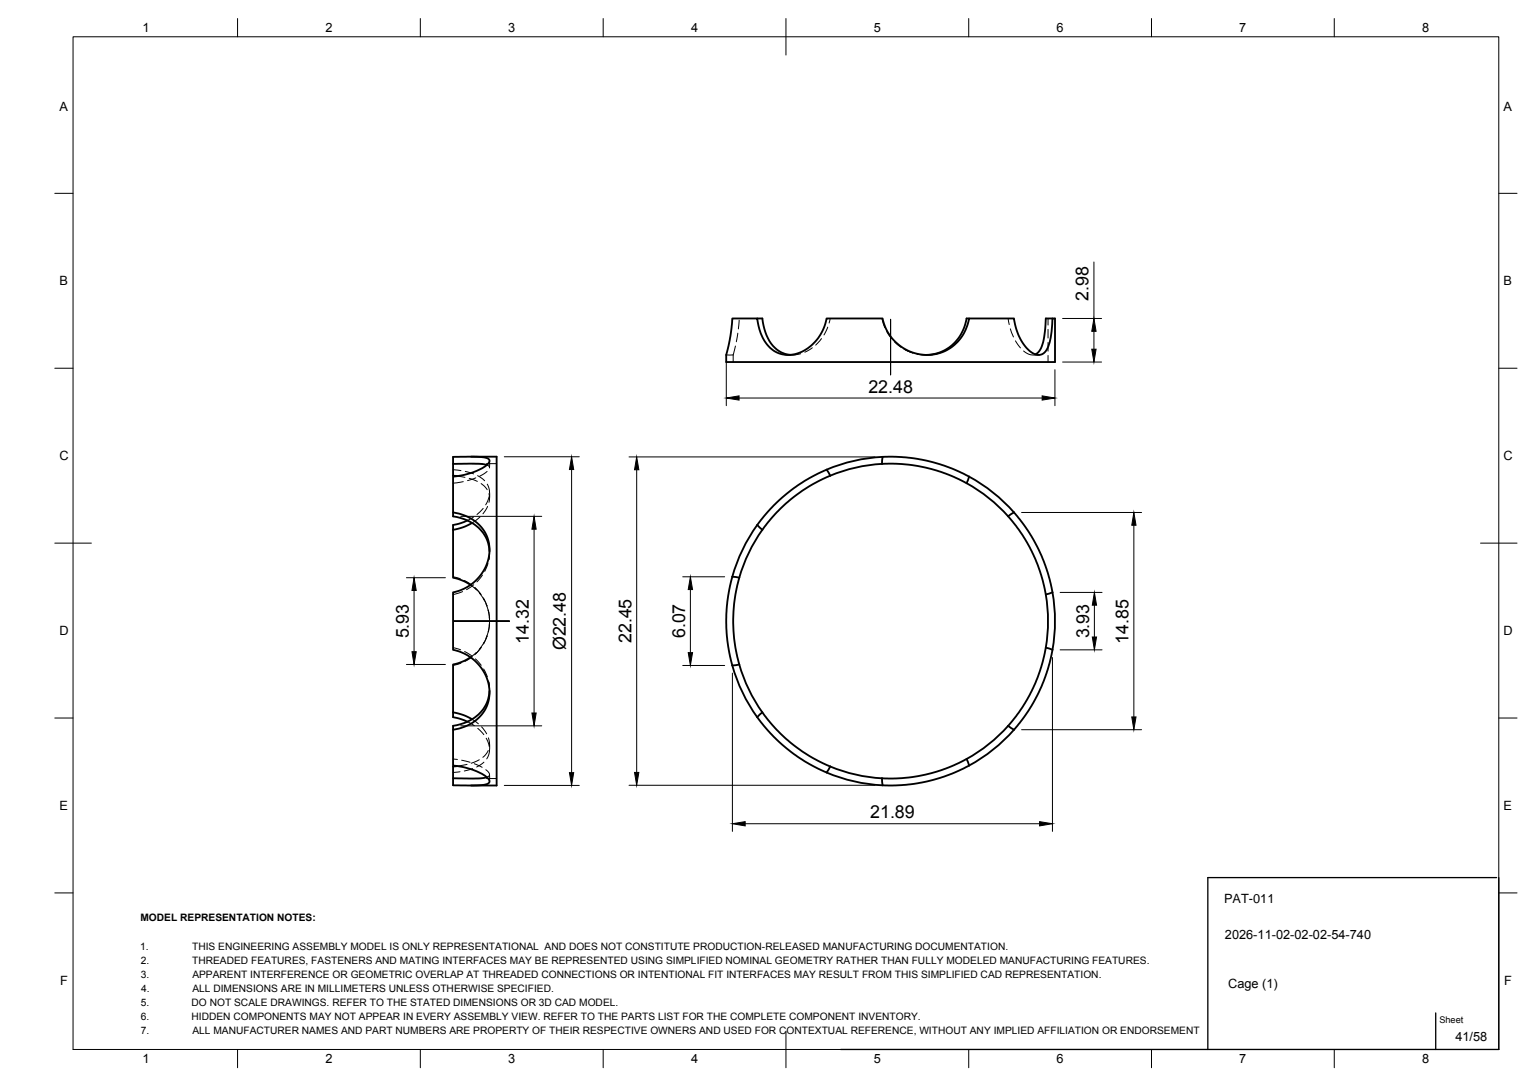
ISO-10303-21;
HEADER;
/* Generated by software containing ST-Developer
 * from STEP Tools, Inc. (www.steptools.com) 
 */

FILE_DESCRIPTION(
/* description */ ('Belt tension measurement rig'),
/* implementation_level */ '2;1');

FILE_NAME(
/* name */ 'Cage (1).step',
/* time_stamp */ '2026-10-28T03:24:44-07:00',
/* author */ (''),
/* organization */ (''),
/* preprocessor_version */ 'ST-DEVELOPER v20.2',
/* originating_system */ 'Autodesk Translation Framework v15.17.0.0',
/* authorisation */ '');

FILE_SCHEMA (('AUTOMOTIVE_DESIGN { 1 0 10303 214 3 1 1 }'));
ENDSEC;

DATA;
#10=MECHANICAL_DESIGN_GEOMETRIC_PRESENTATION_REPRESENTATION('',(#740),#23587);
#460=SPHERICAL_SURFACE('',#13710,0.309556);
#461=SPHERICAL_SURFACE('',#13726,0.309556);
#462=SPHERICAL_SURFACE('',#13731,0.309556);
#463=SPHERICAL_SURFACE('',#13737,0.309556);
#464=SPHERICAL_SURFACE('',#13742,0.309556);
#465=SPHERICAL_SURFACE('',#13747,0.309556);
#466=SPHERICAL_SURFACE('',#13755,0.309556);
#517=B_SPLINE_CURVE_WITH_KNOTS('',3,(#20953,#20954,#20955,#20956,#20957,
#20958,#20959,#20960,#20961,#20962,#20963,#20964,#20965,#20966,#20967,#20968,
#20969,#20970,#20971,#20972,#20973,#20974),.UNSPECIFIED.,.F.,.F.,(4,2,2,
2,2,2,2,2,2,2,4),(0.0591825211272536,0.157966726598481,0.236950089897721,
0.315933453196962,0.391576304923761,0.46721915665056,0.54286200837736,0.618504860104159,
0.697488223403399,0.77647158670264,0.875255792173867),.UNSPECIFIED.);
#518=B_SPLINE_CURVE_WITH_KNOTS('',3,(#20978,#20979,#20980,#20981,#20982,
#20983,#20984,#20985,#20986,#20987,#20988,#20989,#20990,#20991,#20992,#20993,
#20994,#20995,#20996,#20997,#20998,#20999),.UNSPECIFIED.,.F.,.F.,(4,2,2,
2,2,2,2,2,2,2,4),(0.0581119756758434,0.106553146291161,0.213106292582322,
0.30849933801665,0.386091982889075,0.4636846277615,0.541277272633925,0.61886991750635,
0.714262962940678,0.820816109231839,0.869257279847157),.UNSPECIFIED.);
#519=B_SPLINE_CURVE_WITH_KNOTS('',3,(#21005,#21006,#21007,#21008,#21009,
#21010,#21011,#21012,#21013,#21014,#21015,#21016,#21017,#21018,#21019,#21020,
#21021,#21022,#21023,#21024,#21025,#21026),.UNSPECIFIED.,.F.,.F.,(4,2,2,
2,2,2,2,2,2,2,4),(0.0581119756758434,0.106553146291161,0.213106292582322,
0.30849933801665,0.386091982889075,0.4636846277615,0.541277272633925,0.61886991750635,
0.714262962940679,0.820816109231839,0.869257279847157),.UNSPECIFIED.);
#520=B_SPLINE_CURVE_WITH_KNOTS('',3,(#21030,#21031,#21032,#21033,#21034,
#21035,#21036,#21037,#21038,#21039,#21040,#21041,#21042,#21043,#21044,#21045,
#21046,#21047,#21048,#21049,#21050,#21051),.UNSPECIFIED.,.F.,.F.,(4,2,2,
2,2,2,2,2,2,2,4),(0.0581119756758433,0.106553146291161,0.213106292582322,
0.308499338016649,0.386091982889075,0.4636846277615,0.541277272633925,0.61886991750635,
0.714262962940678,0.820816109231839,0.869257279847157),.UNSPECIFIED.);
#521=B_SPLINE_CURVE_WITH_KNOTS('',3,(#21060,#21061,#21062,#21063,#21064,
#21065,#21066,#21067,#21068,#21069,#21070,#21071,#21072,#21073,#21074,#21075,
#21076,#21077,#21078,#21079,#21080,#21081),.UNSPECIFIED.,.F.,.F.,(4,2,2,
2,2,2,2,2,2,2,4),(0.0581119756758433,0.106553146291161,0.213106292582322,
0.30849933801665,0.386091982889075,0.4636846277615,0.541277272633925,0.61886991750635,
0.714262962940678,0.820816109231839,0.869257279847157),.UNSPECIFIED.);
#522=B_SPLINE_CURVE_WITH_KNOTS('',3,(#21085,#21086,#21087,#21088,#21089,
#21090,#21091,#21092,#21093,#21094,#21095,#21096,#21097,#21098,#21099,#21100,
#21101,#21102,#21103,#21104,#21105,#21106),.UNSPECIFIED.,.F.,.F.,(4,2,2,
2,2,2,2,2,2,2,4),(0.0581119756758434,0.106553146291161,0.213106292582322,
0.30849933801665,0.386091982889075,0.4636846277615,0.541277272633925,0.61886991750635,
0.714262962940678,0.820816109231839,0.869257279847157),.UNSPECIFIED.);
#523=B_SPLINE_CURVE_WITH_KNOTS('',3,(#21110,#21111,#21112,#21113,#21114,
#21115,#21116,#21117,#21118,#21119,#21120,#21121,#21122,#21123,#21124,#21125,
#21126,#21127,#21128,#21129,#21130,#21131),.UNSPECIFIED.,.F.,.F.,(4,2,2,
2,2,2,2,2,2,2,4),(0.0581119756758434,0.106553146291161,0.213106292582322,
0.30849933801665,0.386091982889075,0.4636846277615,0.541277272633925,0.61886991750635,
0.714262962940678,0.820816109231839,0.869257279847157),.UNSPECIFIED.);
#524=B_SPLINE_CURVE_WITH_KNOTS('',3,(#21135,#21136,#21137,#21138,#21139,
#21140,#21141,#21142,#21143,#21144,#21145,#21146,#21147,#21148,#21149,#21150,
#21151,#21152,#21153,#21154,#21155,#21156),.UNSPECIFIED.,.F.,.F.,(4,2,2,
2,2,2,2,2,2,2,4),(0.0581119756758433,0.106553146291161,0.213106292582322,
0.30849933801665,0.386091982889075,0.4636846277615,0.541277272633925,0.61886991750635,
0.714262962940678,0.820816109231839,0.869257279847157),.UNSPECIFIED.);
#525=B_SPLINE_CURVE_WITH_KNOTS('',3,(#21164,#21165,#21166,#21167,#21168,
#21169,#21170,#21171,#21172,#21173,#21174,#21175,#21176,#21177,#21178,#21179,
#21180,#21181,#21182,#21183,#21184,#21185),.UNSPECIFIED.,.F.,.F.,(4,2,2,
2,2,2,2,2,2,2,4),(0.0591825211272536,0.157966726598481,0.236950089897721,
0.315933453196962,0.391576304923761,0.467219156650561,0.54286200837736,
0.618504860104159,0.697488223403399,0.77647158670264,0.875255792173867),
 .UNSPECIFIED.);
#526=B_SPLINE_CURVE_WITH_KNOTS('',3,(#21193,#21194,#21195,#21196,#21197,
#21198,#21199,#21200,#21201,#21202,#21203,#21204,#21205,#21206,#21207,#21208,
#21209,#21210,#21211,#21212,#21213,#21214),.UNSPECIFIED.,.F.,.F.,(4,2,2,
2,2,2,2,2,2,2,4),(0.0591825211272536,0.157966726598481,0.236950089897722,
0.315933453196962,0.391576304923761,0.467219156650561,0.54286200837736,
0.618504860104159,0.697488223403399,0.77647158670264,0.875255792173867),
 .UNSPECIFIED.);
#527=B_SPLINE_CURVE_WITH_KNOTS('',3,(#21224,#21225,#21226,#21227,#21228,
#21229,#21230,#21231,#21232,#21233,#21234,#21235,#21236,#21237,#21238,#21239,
#21240,#21241,#21242,#21243,#21244,#21245),.UNSPECIFIED.,.F.,.F.,(4,2,2,
2,2,2,2,2,2,2,4),(0.0591825211272536,0.157966726598481,0.236950089897721,
0.315933453196962,0.391576304923761,0.46721915665056,0.54286200837736,0.618504860104159,
0.697488223403399,0.77647158670264,0.875255792173867),.UNSPECIFIED.);
#528=B_SPLINE_CURVE_WITH_KNOTS('',3,(#21253,#21254,#21255,#21256,#21257,
#21258,#21259,#21260,#21261,#21262,#21263,#21264,#21265,#21266,#21267,#21268,
#21269,#21270,#21271,#21272,#21273,#21274),.UNSPECIFIED.,.F.,.F.,(4,2,2,
2,2,2,2,2,2,2,4),(0.0591825211272536,0.157966726598481,0.236950089897721,
0.315933453196962,0.391576304923761,0.46721915665056,0.542862008377359,
0.618504860104159,0.697488223403399,0.776471586702639,0.875255792173867),
 .UNSPECIFIED.);
#529=B_SPLINE_CURVE_WITH_KNOTS('',3,(#21282,#21283,#21284,#21285,#21286,
#21287,#21288,#21289,#21290,#21291,#21292,#21293,#21294,#21295,#21296,#21297,
#21298,#21299,#21300,#21301,#21302,#21303),.UNSPECIFIED.,.F.,.F.,(4,2,2,
2,2,2,2,2,2,2,4),(0.0591825211272536,0.157966726598481,0.236950089897721,
0.315933453196962,0.391576304923761,0.46721915665056,0.54286200837736,0.618504860104159,
0.697488223403399,0.77647158670264,0.875255792173867),.UNSPECIFIED.);
#530=B_SPLINE_CURVE_WITH_KNOTS('',3,(#21312,#21313,#21314,#21315,#21316,
#21317,#21318,#21319,#21320,#21321,#21322,#21323,#21324,#21325,#21326,#21327,
#21328,#21329,#21330,#21331,#21332,#21333),.UNSPECIFIED.,.F.,.F.,(4,2,2,
2,2,2,2,2,2,2,4),(0.0591825211272536,0.157966726598481,0.236950089897721,
0.315933453196962,0.391576304923761,0.46721915665056,0.542862008377359,
0.618504860104159,0.697488223403399,0.776471586702639,0.875255792173867),
 .UNSPECIFIED.);
#616=SHAPE_REPRESENTATION_RELATIONSHIP('SRR','None',#23865,#671);
#671=ADVANCED_BREP_SHAPE_REPRESENTATION('',(#809),#23563);
#740=STYLED_ITEM('',(#24211),#809);
#809=MANIFOLD_SOLID_BREP('Continuous crown cage',#12246);
#978=FACE_BOUND('',#2627,.T.);
#1254=PLANE('',#13723);
#1255=PLANE('',#13728);
#1256=PLANE('',#13733);
#1257=PLANE('',#13739);
#1258=PLANE('',#13744);
#1259=PLANE('',#13753);
#1260=PLANE('',#13757);
#1261=PLANE('',#13758);
#1758=FACE_OUTER_BOUND('',#2611,.T.);
#1759=FACE_OUTER_BOUND('',#2612,.T.);
#1760=FACE_OUTER_BOUND('',#2613,.T.);
#1761=FACE_OUTER_BOUND('',#2614,.T.);
#1762=FACE_OUTER_BOUND('',#2615,.T.);
#1763=FACE_OUTER_BOUND('',#2616,.T.);
#1764=FACE_OUTER_BOUND('',#2617,.T.);
#1765=FACE_OUTER_BOUND('',#2618,.T.);
#1766=FACE_OUTER_BOUND('',#2619,.T.);
#1767=FACE_OUTER_BOUND('',#2620,.T.);
#1768=FACE_OUTER_BOUND('',#2621,.T.);
#1769=FACE_OUTER_BOUND('',#2622,.T.);
#1770=FACE_OUTER_BOUND('',#2623,.T.);
#1771=FACE_OUTER_BOUND('',#2624,.T.);
#1772=FACE_OUTER_BOUND('',#2625,.T.);
#1773=FACE_OUTER_BOUND('',#2626,.T.);
#1774=FACE_OUTER_BOUND('',#2628,.T.);
#2611=EDGE_LOOP('',(#9740,#9741,#9742,#9743));
#2612=EDGE_LOOP('',(#9744,#9745,#9746,#9747,#9748,#9749,#9750,#9751,#9752,
#9753,#9754,#9755,#9756,#9757,#9758,#9759,#9760,#9761));
#2613=EDGE_LOOP('',(#9762,#9763,#9764,#9765));
#2614=EDGE_LOOP('',(#9766,#9767,#9768,#9769));
#2615=EDGE_LOOP('',(#9770,#9771,#9772,#9773));
#2616=EDGE_LOOP('',(#9774,#9775,#9776,#9777));
#2617=EDGE_LOOP('',(#9778,#9779,#9780,#9781,#9782,#9783));
#2618=EDGE_LOOP('',(#9784,#9785,#9786,#9787));
#2619=EDGE_LOOP('',(#9788,#9789,#9790,#9791));
#2620=EDGE_LOOP('',(#9792,#9793,#9794,#9795));
#2621=EDGE_LOOP('',(#9796,#9797,#9798,#9799));
#2622=EDGE_LOOP('',(#9800,#9801,#9802,#9803));
#2623=EDGE_LOOP('',(#9804,#9805,#9806,#9807,#9808,#9809,#9810,#9811,#9812,
#9813,#9814,#9815,#9816,#9817,#9818,#9819,#9820,#9821));
#2624=EDGE_LOOP('',(#9822,#9823,#9824,#9825));
#2625=EDGE_LOOP('',(#9826,#9827,#9828,#9829));
#2626=EDGE_LOOP('',(#9830));
#2627=EDGE_LOOP('',(#9831));
#2628=EDGE_LOOP('',(#9832,#9833,#9834,#9835));
#3464=LINE('',#21055,#4215);
#3465=LINE('',#21308,#4216);
#4215=VECTOR('',#16695,1.123812);
#4216=VECTOR('',#16764,1.076188);
#4849=CIRCLE('',#13711,0.303778037777585);
#4850=CIRCLE('',#13712,0.303778037777585);
#4851=CIRCLE('',#13714,1.123812);
#4852=CIRCLE('',#13715,1.123812);
#4853=CIRCLE('',#13716,1.123812);
#4854=CIRCLE('',#13717,1.123812);
#4855=CIRCLE('',#13718,1.123812);
#4856=CIRCLE('',#13719,1.123812);
#4857=CIRCLE('',#13720,1.123812);
#4858=CIRCLE('',#13721,1.123812);
#4859=CIRCLE('',#13722,1.123812);
#4860=CIRCLE('',#13724,1.076188);
#4861=CIRCLE('',#13725,0.303778037777585);
#4862=CIRCLE('',#13727,0.303778037777585);
#4863=CIRCLE('',#13729,1.076188);
#4864=CIRCLE('',#13730,0.303778037777585);
#4865=CIRCLE('',#13732,0.303778037777585);
#4866=CIRCLE('',#13734,1.076188);
#4867=CIRCLE('',#13735,1.076188);
#4868=CIRCLE('',#13736,0.303778037777585);
#4869=CIRCLE('',#13738,0.303778037777585);
#4870=CIRCLE('',#13740,1.076188);
#4871=CIRCLE('',#13741,0.303778037777585);
#4872=CIRCLE('',#13743,0.303778037777585);
#4873=CIRCLE('',#13745,1.076188);
#4874=CIRCLE('',#13746,0.303778037777585);
#4875=CIRCLE('',#13748,0.303778037777585);
#4876=CIRCLE('',#13750,1.076188);
#4877=CIRCLE('',#13751,1.076188);
#4878=CIRCLE('',#13752,1.076188);
#4879=CIRCLE('',#13754,0.303778037777585);
#4880=CIRCLE('',#13756,0.303778037777585);
#5852=VERTEX_POINT('',#20951);
#5853=VERTEX_POINT('',#20952);
#5854=VERTEX_POINT('',#20975);
#5855=VERTEX_POINT('',#20977);
#5856=VERTEX_POINT('',#21002);
#5857=VERTEX_POINT('',#21004);
#5858=VERTEX_POINT('',#21027);
#5859=VERTEX_POINT('',#21029);
#5860=VERTEX_POINT('',#21052);
#5861=VERTEX_POINT('',#21054);
#5862=VERTEX_POINT('',#21057);
#5863=VERTEX_POINT('',#21059);
#5864=VERTEX_POINT('',#21082);
#5865=VERTEX_POINT('',#21084);
#5866=VERTEX_POINT('',#21107);
#5867=VERTEX_POINT('',#21109);
#5868=VERTEX_POINT('',#21132);
#5869=VERTEX_POINT('',#21134);
#5870=VERTEX_POINT('',#21159);
#5871=VERTEX_POINT('',#21163);
#5872=VERTEX_POINT('',#21188);
#5873=VERTEX_POINT('',#21192);
#5874=VERTEX_POINT('',#21217);
#5875=VERTEX_POINT('',#21219);
#5876=VERTEX_POINT('',#21223);
#5877=VERTEX_POINT('',#21248);
#5878=VERTEX_POINT('',#21252);
#5879=VERTEX_POINT('',#21277);
#5880=VERTEX_POINT('',#21281);
#5881=VERTEX_POINT('',#21306);
#5882=VERTEX_POINT('',#21309);
#5883=VERTEX_POINT('',#21311);
#7229=EDGE_CURVE('',#5852,#5853,#517,.T.);
#7230=EDGE_CURVE('',#5854,#5852,#4849,.T.);
#7231=EDGE_CURVE('',#5855,#5854,#518,.T.);
#7232=EDGE_CURVE('',#5853,#5855,#4850,.T.);
#7233=EDGE_CURVE('',#5856,#5854,#4851,.T.);
#7234=EDGE_CURVE('',#5856,#5857,#519,.T.);
#7235=EDGE_CURVE('',#5858,#5857,#4852,.T.);
#7236=EDGE_CURVE('',#5858,#5859,#520,.T.);
#7237=EDGE_CURVE('',#5860,#5859,#4853,.T.);
#7238=EDGE_CURVE('',#5860,#5861,#3464,.T.);
#7239=EDGE_CURVE('',#5861,#5861,#4854,.T.);
#7240=EDGE_CURVE('',#5862,#5860,#4855,.T.);
#7241=EDGE_CURVE('',#5862,#5863,#521,.T.);
#7242=EDGE_CURVE('',#5864,#5863,#4856,.T.);
#7243=EDGE_CURVE('',#5864,#5865,#522,.T.);
#7244=EDGE_CURVE('',#5866,#5865,#4857,.T.);
#7245=EDGE_CURVE('',#5866,#5867,#523,.T.);
#7246=EDGE_CURVE('',#5868,#5867,#4858,.T.);
#7247=EDGE_CURVE('',#5868,#5869,#524,.T.);
#7248=EDGE_CURVE('',#5855,#5869,#4859,.T.);
#7249=EDGE_CURVE('',#5852,#5870,#4860,.T.);
#7250=EDGE_CURVE('',#5870,#5856,#4861,.T.);
#7251=EDGE_CURVE('',#5871,#5870,#525,.T.);
#7252=EDGE_CURVE('',#5857,#5871,#4862,.T.);
#7253=EDGE_CURVE('',#5871,#5872,#4863,.T.);
#7254=EDGE_CURVE('',#5872,#5858,#4864,.T.);
#7255=EDGE_CURVE('',#5873,#5872,#526,.T.);
#7256=EDGE_CURVE('',#5859,#5873,#4865,.T.);
#7257=EDGE_CURVE('',#5873,#5874,#4866,.T.);
#7258=EDGE_CURVE('',#5874,#5875,#4867,.T.);
#7259=EDGE_CURVE('',#5875,#5862,#4868,.T.);
#7260=EDGE_CURVE('',#5876,#5875,#527,.T.);
#7261=EDGE_CURVE('',#5863,#5876,#4869,.T.);
#7262=EDGE_CURVE('',#5876,#5877,#4870,.T.);
#7263=EDGE_CURVE('',#5877,#5864,#4871,.T.);
#7264=EDGE_CURVE('',#5878,#5877,#528,.T.);
#7265=EDGE_CURVE('',#5865,#5878,#4872,.T.);
#7266=EDGE_CURVE('',#5878,#5879,#4873,.T.);
#7267=EDGE_CURVE('',#5879,#5866,#4874,.T.);
#7268=EDGE_CURVE('',#5880,#5879,#529,.T.);
#7269=EDGE_CURVE('',#5867,#5880,#4875,.T.);
#7270=EDGE_CURVE('',#5881,#5881,#4876,.T.);
#7271=EDGE_CURVE('',#5881,#5874,#3465,.T.);
#7272=EDGE_CURVE('',#5882,#5853,#4877,.T.);
#7273=EDGE_CURVE('',#5882,#5883,#530,.T.);
#7274=EDGE_CURVE('',#5880,#5883,#4878,.T.);
#7275=EDGE_CURVE('',#5869,#5882,#4879,.T.);
#7276=EDGE_CURVE('',#5883,#5868,#4880,.T.);
#9740=ORIENTED_EDGE('',*,*,#7229,.F.);
#9741=ORIENTED_EDGE('',*,*,#7230,.F.);
#9742=ORIENTED_EDGE('',*,*,#7231,.F.);
#9743=ORIENTED_EDGE('',*,*,#7232,.F.);
#9744=ORIENTED_EDGE('',*,*,#7231,.T.);
#9745=ORIENTED_EDGE('',*,*,#7233,.F.);
#9746=ORIENTED_EDGE('',*,*,#7234,.T.);
#9747=ORIENTED_EDGE('',*,*,#7235,.F.);
#9748=ORIENTED_EDGE('',*,*,#7236,.T.);
#9749=ORIENTED_EDGE('',*,*,#7237,.F.);
#9750=ORIENTED_EDGE('',*,*,#7238,.T.);
#9751=ORIENTED_EDGE('',*,*,#7239,.F.);
#9752=ORIENTED_EDGE('',*,*,#7238,.F.);
#9753=ORIENTED_EDGE('',*,*,#7240,.F.);
#9754=ORIENTED_EDGE('',*,*,#7241,.T.);
#9755=ORIENTED_EDGE('',*,*,#7242,.F.);
#9756=ORIENTED_EDGE('',*,*,#7243,.T.);
#9757=ORIENTED_EDGE('',*,*,#7244,.F.);
#9758=ORIENTED_EDGE('',*,*,#7245,.T.);
#9759=ORIENTED_EDGE('',*,*,#7246,.F.);
#9760=ORIENTED_EDGE('',*,*,#7247,.T.);
#9761=ORIENTED_EDGE('',*,*,#7248,.F.);
#9762=ORIENTED_EDGE('',*,*,#7230,.T.);
#9763=ORIENTED_EDGE('',*,*,#7249,.T.);
#9764=ORIENTED_EDGE('',*,*,#7250,.T.);
#9765=ORIENTED_EDGE('',*,*,#7233,.T.);
#9766=ORIENTED_EDGE('',*,*,#7251,.F.);
#9767=ORIENTED_EDGE('',*,*,#7252,.F.);
#9768=ORIENTED_EDGE('',*,*,#7234,.F.);
#9769=ORIENTED_EDGE('',*,*,#7250,.F.);
#9770=ORIENTED_EDGE('',*,*,#7252,.T.);
#9771=ORIENTED_EDGE('',*,*,#7253,.T.);
#9772=ORIENTED_EDGE('',*,*,#7254,.T.);
#9773=ORIENTED_EDGE('',*,*,#7235,.T.);
#9774=ORIENTED_EDGE('',*,*,#7255,.F.);
#9775=ORIENTED_EDGE('',*,*,#7256,.F.);
#9776=ORIENTED_EDGE('',*,*,#7236,.F.);
#9777=ORIENTED_EDGE('',*,*,#7254,.F.);
#9778=ORIENTED_EDGE('',*,*,#7256,.T.);
#9779=ORIENTED_EDGE('',*,*,#7257,.T.);
#9780=ORIENTED_EDGE('',*,*,#7258,.T.);
#9781=ORIENTED_EDGE('',*,*,#7259,.T.);
#9782=ORIENTED_EDGE('',*,*,#7240,.T.);
#9783=ORIENTED_EDGE('',*,*,#7237,.T.);
#9784=ORIENTED_EDGE('',*,*,#7260,.F.);
#9785=ORIENTED_EDGE('',*,*,#7261,.F.);
#9786=ORIENTED_EDGE('',*,*,#7241,.F.);
#9787=ORIENTED_EDGE('',*,*,#7259,.F.);
#9788=ORIENTED_EDGE('',*,*,#7261,.T.);
#9789=ORIENTED_EDGE('',*,*,#7262,.T.);
#9790=ORIENTED_EDGE('',*,*,#7263,.T.);
#9791=ORIENTED_EDGE('',*,*,#7242,.T.);
#9792=ORIENTED_EDGE('',*,*,#7264,.F.);
#9793=ORIENTED_EDGE('',*,*,#7265,.F.);
#9794=ORIENTED_EDGE('',*,*,#7243,.F.);
#9795=ORIENTED_EDGE('',*,*,#7263,.F.);
#9796=ORIENTED_EDGE('',*,*,#7265,.T.);
#9797=ORIENTED_EDGE('',*,*,#7266,.T.);
#9798=ORIENTED_EDGE('',*,*,#7267,.T.);
#9799=ORIENTED_EDGE('',*,*,#7244,.T.);
#9800=ORIENTED_EDGE('',*,*,#7245,.F.);
#9801=ORIENTED_EDGE('',*,*,#7267,.F.);
#9802=ORIENTED_EDGE('',*,*,#7268,.F.);
#9803=ORIENTED_EDGE('',*,*,#7269,.F.);
#9804=ORIENTED_EDGE('',*,*,#7270,.F.);
#9805=ORIENTED_EDGE('',*,*,#7271,.T.);
#9806=ORIENTED_EDGE('',*,*,#7257,.F.);
#9807=ORIENTED_EDGE('',*,*,#7255,.T.);
#9808=ORIENTED_EDGE('',*,*,#7253,.F.);
#9809=ORIENTED_EDGE('',*,*,#7251,.T.);
#9810=ORIENTED_EDGE('',*,*,#7249,.F.);
#9811=ORIENTED_EDGE('',*,*,#7229,.T.);
#9812=ORIENTED_EDGE('',*,*,#7272,.F.);
#9813=ORIENTED_EDGE('',*,*,#7273,.T.);
#9814=ORIENTED_EDGE('',*,*,#7274,.F.);
#9815=ORIENTED_EDGE('',*,*,#7268,.T.);
#9816=ORIENTED_EDGE('',*,*,#7266,.F.);
#9817=ORIENTED_EDGE('',*,*,#7264,.T.);
#9818=ORIENTED_EDGE('',*,*,#7262,.F.);
#9819=ORIENTED_EDGE('',*,*,#7260,.T.);
#9820=ORIENTED_EDGE('',*,*,#7258,.F.);
#9821=ORIENTED_EDGE('',*,*,#7271,.F.);
#9822=ORIENTED_EDGE('',*,*,#7232,.T.);
#9823=ORIENTED_EDGE('',*,*,#7248,.T.);
#9824=ORIENTED_EDGE('',*,*,#7275,.T.);
#9825=ORIENTED_EDGE('',*,*,#7272,.T.);
#9826=ORIENTED_EDGE('',*,*,#7247,.F.);
#9827=ORIENTED_EDGE('',*,*,#7276,.F.);
#9828=ORIENTED_EDGE('',*,*,#7273,.F.);
#9829=ORIENTED_EDGE('',*,*,#7275,.F.);
#9830=ORIENTED_EDGE('',*,*,#7239,.T.);
#9831=ORIENTED_EDGE('',*,*,#7270,.T.);
#9832=ORIENTED_EDGE('',*,*,#7269,.T.);
#9833=ORIENTED_EDGE('',*,*,#7274,.T.);
#9834=ORIENTED_EDGE('',*,*,#7276,.T.);
#9835=ORIENTED_EDGE('',*,*,#7246,.T.);
#11309=CYLINDRICAL_SURFACE('',#13713,1.123812);
#11310=CYLINDRICAL_SURFACE('',#13749,1.076188);
#11899=ADVANCED_FACE('',(#1758),#460,.F.);
#11900=ADVANCED_FACE('',(#1759),#11309,.T.);
#11901=ADVANCED_FACE('',(#1760),#1254,.T.);
#11902=ADVANCED_FACE('',(#1761),#461,.F.);
#11903=ADVANCED_FACE('',(#1762),#1255,.T.);
#11904=ADVANCED_FACE('',(#1763),#462,.F.);
#11905=ADVANCED_FACE('',(#1764),#1256,.T.);
#11906=ADVANCED_FACE('',(#1765),#463,.F.);
#11907=ADVANCED_FACE('',(#1766),#1257,.T.);
#11908=ADVANCED_FACE('',(#1767),#464,.F.);
#11909=ADVANCED_FACE('',(#1768),#1258,.T.);
#11910=ADVANCED_FACE('',(#1769),#465,.F.);
#11911=ADVANCED_FACE('',(#1770),#11310,.F.);
#11912=ADVANCED_FACE('',(#1771),#1259,.T.);
#11913=ADVANCED_FACE('',(#1772),#466,.F.);
#11914=ADVANCED_FACE('',(#1773,#978),#1260,.T.);
#11915=ADVANCED_FACE('',(#1774),#1261,.T.);
#12246=CLOSED_SHELL('',(#11899,#11900,#11901,#11902,#11903,#11904,#11905,
#11906,#11907,#11908,#11909,#11910,#11911,#11912,#11913,#11914,#11915));
#13709=AXIS2_PLACEMENT_3D('',#20949,#16679,#16680);
#13710=AXIS2_PLACEMENT_3D('',#20950,#16681,#16682);
#13711=AXIS2_PLACEMENT_3D('',#20976,#16683,#16684);
#13712=AXIS2_PLACEMENT_3D('',#21000,#16685,#16686);
#13713=AXIS2_PLACEMENT_3D('',#21001,#16687,#16688);
#13714=AXIS2_PLACEMENT_3D('',#21003,#16689,#16690);
#13715=AXIS2_PLACEMENT_3D('',#21028,#16691,#16692);
#13716=AXIS2_PLACEMENT_3D('',#21053,#16693,#16694);
#13717=AXIS2_PLACEMENT_3D('',#21056,#16696,#16697);
#13718=AXIS2_PLACEMENT_3D('',#21058,#16698,#16699);
#13719=AXIS2_PLACEMENT_3D('',#21083,#16700,#16701);
#13720=AXIS2_PLACEMENT_3D('',#21108,#16702,#16703);
#13721=AXIS2_PLACEMENT_3D('',#21133,#16704,#16705);
#13722=AXIS2_PLACEMENT_3D('',#21157,#16706,#16707);
#13723=AXIS2_PLACEMENT_3D('',#21158,#16708,#16709);
#13724=AXIS2_PLACEMENT_3D('',#21160,#16710,#16711);
#13725=AXIS2_PLACEMENT_3D('',#21161,#16712,#16713);
#13726=AXIS2_PLACEMENT_3D('',#21162,#16714,#16715);
#13727=AXIS2_PLACEMENT_3D('',#21186,#16716,#16717);
#13728=AXIS2_PLACEMENT_3D('',#21187,#16718,#16719);
#13729=AXIS2_PLACEMENT_3D('',#21189,#16720,#16721);
#13730=AXIS2_PLACEMENT_3D('',#21190,#16722,#16723);
#13731=AXIS2_PLACEMENT_3D('',#21191,#16724,#16725);
#13732=AXIS2_PLACEMENT_3D('',#21215,#16726,#16727);
#13733=AXIS2_PLACEMENT_3D('',#21216,#16728,#16729);
#13734=AXIS2_PLACEMENT_3D('',#21218,#16730,#16731);
#13735=AXIS2_PLACEMENT_3D('',#21220,#16732,#16733);
#13736=AXIS2_PLACEMENT_3D('',#21221,#16734,#16735);
#13737=AXIS2_PLACEMENT_3D('',#21222,#16736,#16737);
#13738=AXIS2_PLACEMENT_3D('',#21246,#16738,#16739);
#13739=AXIS2_PLACEMENT_3D('',#21247,#16740,#16741);
#13740=AXIS2_PLACEMENT_3D('',#21249,#16742,#16743);
#13741=AXIS2_PLACEMENT_3D('',#21250,#16744,#16745);
#13742=AXIS2_PLACEMENT_3D('',#21251,#16746,#16747);
#13743=AXIS2_PLACEMENT_3D('',#21275,#16748,#16749);
#13744=AXIS2_PLACEMENT_3D('',#21276,#16750,#16751);
#13745=AXIS2_PLACEMENT_3D('',#21278,#16752,#16753);
#13746=AXIS2_PLACEMENT_3D('',#21279,#16754,#16755);
#13747=AXIS2_PLACEMENT_3D('',#21280,#16756,#16757);
#13748=AXIS2_PLACEMENT_3D('',#21304,#16758,#16759);
#13749=AXIS2_PLACEMENT_3D('',#21305,#16760,#16761);
#13750=AXIS2_PLACEMENT_3D('',#21307,#16762,#16763);
#13751=AXIS2_PLACEMENT_3D('',#21310,#16765,#16766);
#13752=AXIS2_PLACEMENT_3D('',#21334,#16767,#16768);
#13753=AXIS2_PLACEMENT_3D('',#21335,#16769,#16770);
#13754=AXIS2_PLACEMENT_3D('',#21336,#16771,#16772);
#13755=AXIS2_PLACEMENT_3D('',#21337,#16773,#16774);
#13756=AXIS2_PLACEMENT_3D('',#21338,#16775,#16776);
#13757=AXIS2_PLACEMENT_3D('',#21339,#16777,#16778);
#13758=AXIS2_PLACEMENT_3D('',#21340,#16779,#16780);
#16679=DIRECTION('axis',(0.,0.,1.));
#16680=DIRECTION('refdir',(1.,0.,0.));
#16681=DIRECTION('center_axis',(0.,0.,1.));
#16682=DIRECTION('ref_axis',(1.,0.,0.));
#16683=DIRECTION('center_axis',(0.,-1.,0.));
#16684=DIRECTION('ref_axis',(0.,0.,-1.));
#16685=DIRECTION('center_axis',(0.,-1.,0.));
#16686=DIRECTION('ref_axis',(0.,0.,-1.));
#16687=DIRECTION('center_axis',(0.,1.,0.));
#16688=DIRECTION('ref_axis',(1.,0.,0.));
#16689=DIRECTION('center_axis',(0.,1.,0.));
#16690=DIRECTION('ref_axis',(1.,0.,0.));
#16691=DIRECTION('center_axis',(0.,1.,0.));
#16692=DIRECTION('ref_axis',(1.,0.,0.));
#16693=DIRECTION('center_axis',(0.,1.,0.));
#16694=DIRECTION('ref_axis',(1.,0.,0.));
#16695=DIRECTION('',(0.,-1.,0.));
#16696=DIRECTION('center_axis',(0.,-1.,0.));
#16697=DIRECTION('ref_axis',(1.,0.,0.));
#16698=DIRECTION('center_axis',(0.,1.,0.));
#16699=DIRECTION('ref_axis',(1.,0.,0.));
#16700=DIRECTION('center_axis',(0.,1.,0.));
#16701=DIRECTION('ref_axis',(1.,0.,0.));
#16702=DIRECTION('center_axis',(0.,1.,0.));
#16703=DIRECTION('ref_axis',(1.,0.,0.));
#16704=DIRECTION('center_axis',(0.,1.,0.));
#16705=DIRECTION('ref_axis',(1.,0.,0.));
#16706=DIRECTION('center_axis',(0.,1.,0.));
#16707=DIRECTION('ref_axis',(1.,0.,0.));
#16708=DIRECTION('center_axis',(0.,1.,0.));
#16709=DIRECTION('ref_axis',(1.,0.,0.));
#16710=DIRECTION('center_axis',(0.,-1.,0.));
#16711=DIRECTION('ref_axis',(1.,0.,0.));
#16712=DIRECTION('center_axis',(0.,-1.,0.));
#16713=DIRECTION('ref_axis',(0.,0.,-1.));
#16714=DIRECTION('center_axis',(8.96625347776458E-17,0.,1.));
#16715=DIRECTION('ref_axis',(1.,0.,0.));
#16716=DIRECTION('center_axis',(0.,-1.,0.));
#16717=DIRECTION('ref_axis',(0.,0.,-1.));
#16718=DIRECTION('center_axis',(0.,1.,0.));
#16719=DIRECTION('ref_axis',(1.,0.,0.));
#16720=DIRECTION('center_axis',(0.,-1.,0.));
#16721=DIRECTION('ref_axis',(1.,0.,0.));
#16722=DIRECTION('center_axis',(0.,-1.,0.));
#16723=DIRECTION('ref_axis',(0.,0.,-1.));
#16724=DIRECTION('center_axis',(0.,0.,1.));
#16725=DIRECTION('ref_axis',(1.,0.,0.));
#16726=DIRECTION('center_axis',(0.,-1.,0.));
#16727=DIRECTION('ref_axis',(0.,0.,-1.));
#16728=DIRECTION('center_axis',(0.,1.,0.));
#16729=DIRECTION('ref_axis',(1.,0.,0.));
#16730=DIRECTION('center_axis',(0.,-1.,0.));
#16731=DIRECTION('ref_axis',(1.,0.,0.));
#16732=DIRECTION('center_axis',(0.,-1.,0.));
#16733=DIRECTION('ref_axis',(1.,0.,0.));
#16734=DIRECTION('center_axis',(0.,-1.,0.));
#16735=DIRECTION('ref_axis',(0.,0.,-1.));
#16736=DIRECTION('center_axis',(0.,0.,1.));
#16737=DIRECTION('ref_axis',(1.,0.,0.));
#16738=DIRECTION('center_axis',(0.,-1.,0.));
#16739=DIRECTION('ref_axis',(0.,0.,-1.));
#16740=DIRECTION('center_axis',(0.,1.,0.));
#16741=DIRECTION('ref_axis',(1.,0.,0.));
#16742=DIRECTION('center_axis',(0.,-1.,0.));
#16743=DIRECTION('ref_axis',(1.,0.,0.));
#16744=DIRECTION('center_axis',(0.,-1.,0.));
#16745=DIRECTION('ref_axis',(0.,0.,-1.));
#16746=DIRECTION('center_axis',(8.96625347776458E-17,0.,1.));
#16747=DIRECTION('ref_axis',(1.,0.,0.));
#16748=DIRECTION('center_axis',(0.,-1.,0.));
#16749=DIRECTION('ref_axis',(0.,0.,-1.));
#16750=DIRECTION('center_axis',(0.,1.,0.));
#16751=DIRECTION('ref_axis',(1.,0.,0.));
#16752=DIRECTION('center_axis',(0.,-1.,0.));
#16753=DIRECTION('ref_axis',(1.,0.,0.));
#16754=DIRECTION('center_axis',(0.,-1.,0.));
#16755=DIRECTION('ref_axis',(0.,0.,-1.));
#16756=DIRECTION('center_axis',(0.,0.,1.));
#16757=DIRECTION('ref_axis',(1.,0.,0.));
#16758=DIRECTION('center_axis',(0.,-1.,0.));
#16759=DIRECTION('ref_axis',(0.,0.,-1.));
#16760=DIRECTION('center_axis',(0.,1.,0.));
#16761=DIRECTION('ref_axis',(1.,0.,0.));
#16762=DIRECTION('center_axis',(0.,1.,0.));
#16763=DIRECTION('ref_axis',(1.,0.,0.));
#16764=DIRECTION('',(0.,1.,0.));
#16765=DIRECTION('center_axis',(0.,-1.,0.));
#16766=DIRECTION('ref_axis',(1.,0.,0.));
#16767=DIRECTION('center_axis',(0.,-1.,0.));
#16768=DIRECTION('ref_axis',(1.,0.,0.));
#16769=DIRECTION('center_axis',(0.,1.,0.));
#16770=DIRECTION('ref_axis',(1.,0.,0.));
#16771=DIRECTION('center_axis',(0.,-1.,0.));
#16772=DIRECTION('ref_axis',(0.,0.,-1.));
#16773=DIRECTION('center_axis',(0.,0.,1.));
#16774=DIRECTION('ref_axis',(1.,0.,0.));
#16775=DIRECTION('center_axis',(0.,-1.,0.));
#16776=DIRECTION('ref_axis',(0.,0.,-1.));
#16777=DIRECTION('center_axis',(0.,-1.,0.));
#16778=DIRECTION('ref_axis',(-1.,0.,0.));
#16779=DIRECTION('center_axis',(0.,1.,0.));
#16780=DIRECTION('ref_axis',(1.,0.,0.));
#20949=CARTESIAN_POINT('',(0.,0.,0.));
#20950=CARTESIAN_POINT('Origin',(0.685838782044607,0.,0.860014630714833));
#20951=CARTESIAN_POINT('',(0.413083465285518,-0.05953,0.993751811093549));
#20952=CARTESIAN_POINT('',(0.876916659919095,-0.05953,0.623857181492959));
#20953=CARTESIAN_POINT('Ctrl Pts',(0.413083465285518,-0.05953,0.993751811093549));
#20954=CARTESIAN_POINT('Ctrl Pts',(0.419070565453383,-0.0925528133349865,
0.991263089003441));
#20955=CARTESIAN_POINT('Ctrl Pts',(0.430199341854858,-0.124911173756694,
0.986608710139579));
#20956=CARTESIAN_POINT('Ctrl Pts',(0.457978755888596,-0.177924977804098,
0.973971221090534));
#20957=CARTESIAN_POINT('Ctrl Pts',(0.473077587363685,-0.199697230012983,
0.966820759530997));
#20958=CARTESIAN_POINT('Ctrl Pts',(0.507057380724533,-0.237895043532788,
0.949440676105255));
#20959=CARTESIAN_POINT('Ctrl Pts',(0.525933334162555,-0.254319232363049,
0.939198248544428));
#20960=CARTESIAN_POINT('Ctrl Pts',(0.564362943424238,-0.28018331644634,
0.916597376014514));
#20961=CARTESIAN_POINT('Ctrl Pts',(0.585840553788742,-0.29104845371857,
0.903141581680914));
#20962=CARTESIAN_POINT('Ctrl Pts',(0.629305439856167,-0.30527573347708,
0.873412008702649));
#20963=CARTESIAN_POINT('Ctrl Pts',(0.651278921914856,-0.308638795020976,
0.857118508332695));
#20964=CARTESIAN_POINT('Ctrl Pts',(0.690705563850638,-0.308638795020976,
0.825676810575914));
#20965=CARTESIAN_POINT('Ctrl Pts',(0.711480111898423,-0.30527573347708,
0.807879894508811));
#20966=CARTESIAN_POINT('Ctrl Pts',(0.750136149454208,-0.29104845371857,
0.772120216227122));
#20967=CARTESIAN_POINT('Ctrl Pts',(0.768033796848072,-0.28018331644634,
0.754175290318038));
#20968=CARTESIAN_POINT('Ctrl Pts',(0.798619410861634,-0.254319232363049,
0.721738358858166));
#20969=CARTESIAN_POINT('Ctrl Pts',(0.812805334167529,-0.237895043532788,
0.705614819529209));
#20970=CARTESIAN_POINT('Ctrl Pts',(0.837310877969633,-0.199697230012983,
0.676354402927683));
#20971=CARTESIAN_POINT('Ctrl Pts',(0.847641868610495,-0.177924977804098,
0.663225258065736));
#20972=CARTESIAN_POINT('Ctrl Pts',(0.866144010579847,-0.124911173756694,
0.638954437806245));
#20973=CARTESIAN_POINT('Ctrl Pts',(0.873158080166742,-0.0925528133349865,
0.62914037979579));
#20974=CARTESIAN_POINT('Ctrl Pts',(0.876916659919095,-0.05953,0.623857181492959));
#20975=CARTESIAN_POINT('',(0.437601487681057,-0.05953,1.03511272300331));
#20976=CARTESIAN_POINT('Origin',(0.685838782044607,-0.05953,0.860014630714833));
#20977=CARTESIAN_POINT('',(0.911784794170997,-0.05953,0.656964154625313));
#20978=CARTESIAN_POINT('Ctrl Pts',(0.911784794170998,-0.0595300000000001,
0.656964154625312));
#20979=CARTESIAN_POINT('Ctrl Pts',(0.909827729890942,-0.0762225747374255,
0.659680317203144));
#20980=CARTESIAN_POINT('Ctrl Pts',(0.907004864562642,-0.0928409665394228,
0.663576540841106));
#20981=CARTESIAN_POINT('Ctrl Pts',(0.895234408667242,-0.144299303100741,
0.679480524217551));
#20982=CARTESIAN_POINT('Ctrl Pts',(0.882797231409153,-0.177024326825049,
0.695831250979106));
#20983=CARTESIAN_POINT('Ctrl Pts',(0.854332839576145,-0.227269801620064,
0.73042219438957));
#20984=CARTESIAN_POINT('Ctrl Pts',(0.834863020612702,-0.251265615809407,
0.752807465209441));
#20985=CARTESIAN_POINT('Ctrl Pts',(0.800439809856111,-0.279889827963178,
0.789147407129766));
#20986=CARTESIAN_POINT('Ctrl Pts',(0.781998747691871,-0.290879136862659,
0.80756613568454));
#20987=CARTESIAN_POINT('Ctrl Pts',(0.742239891936898,-0.305251990234487,
0.844254137480382));
#20988=CARTESIAN_POINT('Ctrl Pts',(0.720906778729541,-0.308638795020976,
0.862505527716294));
#20989=CARTESIAN_POINT('Ctrl Pts',(0.680463863683392,-0.308638795020976,
0.894757676234429));
#20990=CARTESIAN_POINT('Ctrl Pts',(0.657923009631182,-0.305251990234488,
0.91149460735272));
#20991=CARTESIAN_POINT('Ctrl Pts',(0.613307674922609,-0.290879136862659,
0.942092777160053));
#20992=CARTESIAN_POINT('Ctrl Pts',(0.591247219971725,-0.279889827963178,
0.955972930713954));
#20993=CARTESIAN_POINT('Ctrl Pts',(0.548158511259202,-0.251265615809407,
0.981446681891443));
#20994=CARTESIAN_POINT('Ctrl Pts',(0.522002043615455,-0.227269801620063,
0.995447160474328));
#20995=CARTESIAN_POINT('Ctrl Pts',(0.481944444320713,-0.177024326825049,
1.01550068154148));
#20996=CARTESIAN_POINT('Ctrl Pts',(0.463236132117164,-0.14429930310074,
1.0239876538093));
#20997=CARTESIAN_POINT('Ctrl Pts',(0.445111721969657,-0.0928409665394226,
1.03192403056628));
#20998=CARTESIAN_POINT('Ctrl Pts',(0.440685038163619,-0.0762225747374254,
1.03380912944435));
#20999=CARTESIAN_POINT('Ctrl Pts',(0.437601487681056,-0.05953,1.03511272300331));
#21000=CARTESIAN_POINT('Origin',(0.685838782044607,-0.05953,0.860014630714833));
#21001=CARTESIAN_POINT('Origin',(0.,-0.208355,0.));
#21002=CARTESIAN_POINT('',(0.0548532617164168,-0.05953,1.12247250791415));
#21003=CARTESIAN_POINT('Origin',(0.,-0.05953,0.));
#21004=CARTESIAN_POINT('',(-0.536443649899848,-0.05953,0.987512846410683));
#21005=CARTESIAN_POINT('Ctrl Pts',(0.0548532617164173,-0.0595300000000001,
1.12247250791414));
#21006=CARTESIAN_POINT('Ctrl Pts',(0.05150947068137,-0.0762225747374254,
1.12263591311425));
#21007=CARTESIAN_POINT('Ctrl Pts',(0.0467032526342597,-0.0928409665394227,
1.12285816383385));
#21008=CARTESIAN_POINT('Ctrl Pts',(0.0269302585198975,-0.144299303100741,
1.12357162229597));
#21009=CARTESIAN_POINT('Ctrl Pts',(0.006392292392153,-0.177024326825049,
1.12404235695137));
#21010=CARTESIAN_POINT('Ctrl Pts',(-0.0383992541984087,-0.227269801620063,
1.12335509974011));
#21011=CARTESIAN_POINT('Ctrl Pts',(-0.0680399972366993,-0.251265615809407,
1.12208997038458));
#21012=CARTESIAN_POINT('Ctrl Pts',(-0.117914228755037,-0.279889827963178,
1.1178344036749));
#21013=CARTESIAN_POINT('Ctrl Pts',(-0.14381238480104,-0.290879136862659,
1.11490049012186));
#21014=CARTESIAN_POINT('Ctrl Pts',(-0.19728546073067,-0.305251990234488,
1.10669035995599));
#21015=CARTESIAN_POINT('Ctrl Pts',(-0.224855950742601,-0.308638795020976,
1.10139101611326));
#21016=CARTESIAN_POINT('Ctrl Pts',(-0.275287440920027,-0.308638795020976,
1.0898803575765));
#21017=CARTESIAN_POINT('Ctrl Pts',(-0.302426893214945,-0.305251990234488,
1.08269251410343));
#21018=CARTESIAN_POINT('Ctrl Pts',(-0.35416671187353,-0.290879136862659,
1.06688848765783));
#21019=CARTESIAN_POINT('Ctrl Pts',(-0.3787731215897,-0.279889827963178,
1.05829506364875));
#21020=CARTESIAN_POINT('Ctrl Pts',(-0.425554672694338,-0.251265615809407,
1.04048957871266));
#21021=CARTESIAN_POINT('Ctrl Pts',(-0.452808978448581,-0.227269801620063,
1.02876878445619));
#21022=CARTESIAN_POINT('Ctrl Pts',(-0.493462957200432,-0.177024326825049,
1.0099536580922));
#21023=CARTESIAN_POINT('Ctrl Pts',(-0.511762781179148,-0.14429930310074,
1.00061845128527));
#21024=CARTESIAN_POINT('Ctrl Pts',(-0.529268075276157,-0.0928409665394226,
0.991396466802468));
#21025=CARTESIAN_POINT('Ctrl Pts',(-0.533501897135713,-0.0762225747374254,
0.989110885965947));
#21026=CARTESIAN_POINT('Ctrl Pts',(-0.536443649899848,-0.0595300000000001,
0.987512846410683));
#21027=CARTESIAN_POINT('',(-0.843383895613249,-0.05953,0.742736168477219));
#21028=CARTESIAN_POINT('Origin',(0.,-0.05953,0.));
#21029=CARTESIAN_POINT('',(-1.10653577764992,-0.05953,0.196295654879792));
#21030=CARTESIAN_POINT('Ctrl Pts',(-0.843383895613249,-0.0595300000000001,
0.742736168477219));
#21031=CARTESIAN_POINT('Ctrl Pts',(-0.84559647055299,-0.0762225747374255,
0.740223768851062));
#21032=CARTESIAN_POINT('Ctrl Pts',(-0.848766861100456,-0.0928409665394227,
0.736604687327351));
#21033=CARTESIAN_POINT('Ctrl Pts',(-0.861652925570091,-0.144299303100741,
0.721590372101268));
#21034=CARTESIAN_POINT('Ctrl Pts',(-0.87482617317514,-0.177024326825049,
0.705826641853758));
#21035=CARTESIAN_POINT('Ctrl Pts',(-0.902215926359523,-0.227269801620063,
0.670378702718353));
#21036=CARTESIAN_POINT('Ctrl Pts',(-0.919707509403859,-0.251265615809407,
0.646415841396062));
#21037=CARTESIAN_POINT('Ctrl Pts',(-0.947476448101718,-0.279889827963178,
0.604769294586516));
#21038=CARTESIAN_POINT('Ctrl Pts',(-0.961329858300736,-0.290879136862659,
0.582692035672022));
#21039=CARTESIAN_POINT('Ctrl Pts',(-0.988250837578047,-0.305251990234488,
0.535766169015486));
#21040=CARTESIAN_POINT('Ctrl Pts',(-1.00129756308006,-0.308638795020976,
0.510906605094603));
#21041=CARTESIAN_POINT('Ctrl Pts',(-1.02374168767024,-0.308638795020976,
0.46430090015576));
#21042=CARTESIAN_POINT('Ctrl Pts',(-1.03504317708586,-0.305251990234488,
0.438600874831839));
#21043=CARTESIAN_POINT('Ctrl Pts',(-1.05494634094458,-0.290879136862659,
0.388295406390235));
#21044=CARTESIAN_POINT('Ctrl Pts',(-1.06356957703048,-0.279889827963178,
0.363699428370917));
#21045=CARTESIAN_POINT('Ctrl Pts',(-1.0788165083757,-0.251265615809407,
0.316022600643821));
#21046=CARTESIAN_POINT('Ctrl Pts',(-1.08664560412098,-0.227269801620063,
0.287406530683752));
#21047=CARTESIAN_POINT('Ctrl Pts',(-1.09728268713976,-0.177024326825049,
0.243890930799337));
#21048=CARTESIAN_POINT('Ctrl Pts',(-1.10139388218929,-0.144299303100741,
0.22376314604679));
#21049=CARTESIAN_POINT('Ctrl Pts',(-1.10509821673782,-0.0928409665394227,
0.204327142733961));
#21050=CARTESIAN_POINT('Ctrl Pts',(-1.10595102243643,-0.0762225747374254,
0.199591971170104));
#21051=CARTESIAN_POINT('Ctrl Pts',(-1.10653577764992,-0.0595300000000001,
0.196295654879792));
#21052=CARTESIAN_POINT('',(-1.123812,-0.05953,1.37627276864339E-16));
#21053=CARTESIAN_POINT('Origin',(0.,-0.05953,0.));
#21054=CARTESIAN_POINT('',(-1.123812,-0.35718,1.37627276864339E-16));
#21055=CARTESIAN_POINT('',(-1.123812,-0.208355,1.37627276864339E-16));
#21056=CARTESIAN_POINT('Origin',(0.,-0.35718,0.));
#21057=CARTESIAN_POINT('',(-1.10653577764992,-0.05953,-0.196295654879793));
#21058=CARTESIAN_POINT('Origin',(0.,-0.05953,0.));
#21059=CARTESIAN_POINT('',(-0.843383895613249,-0.05953,-0.742736168477219));
#21060=CARTESIAN_POINT('Ctrl Pts',(-1.10653577764992,-0.0595300000000001,
-0.196295654879792));
#21061=CARTESIAN_POINT('Ctrl Pts',(-1.10595102243643,-0.0762225747374255,
-0.199591971170104));
#21062=CARTESIAN_POINT('Ctrl Pts',(-1.10509821673782,-0.0928409665394228,
-0.204327142733962));
#21063=CARTESIAN_POINT('Ctrl Pts',(-1.10139388218929,-0.144299303100741,
-0.22376314604679));
#21064=CARTESIAN_POINT('Ctrl Pts',(-1.09728268713976,-0.177024326825049,
-0.243890930799338));
#21065=CARTESIAN_POINT('Ctrl Pts',(-1.08664560412098,-0.227269801620063,
-0.287406530683753));
#21066=CARTESIAN_POINT('Ctrl Pts',(-1.0788165083757,-0.251265615809407,
-0.316022600643821));
#21067=CARTESIAN_POINT('Ctrl Pts',(-1.06356957703048,-0.279889827963178,
-0.363699428370918));
#21068=CARTESIAN_POINT('Ctrl Pts',(-1.05494634094458,-0.290879136862659,
-0.388295406390235));
#21069=CARTESIAN_POINT('Ctrl Pts',(-1.03504317708586,-0.305251990234488,
-0.438600874831839));
#21070=CARTESIAN_POINT('Ctrl Pts',(-1.02374168767024,-0.308638795020976,
-0.46430090015576));
#21071=CARTESIAN_POINT('Ctrl Pts',(-1.00129756308006,-0.308638795020976,
-0.510906605094603));
#21072=CARTESIAN_POINT('Ctrl Pts',(-0.988250837578047,-0.305251990234488,
-0.535766169015486));
#21073=CARTESIAN_POINT('Ctrl Pts',(-0.961329858300736,-0.290879136862659,
-0.582692035672022));
#21074=CARTESIAN_POINT('Ctrl Pts',(-0.947476448101718,-0.279889827963178,
-0.604769294586516));
#21075=CARTESIAN_POINT('Ctrl Pts',(-0.919707509403859,-0.251265615809407,
-0.646415841396062));
#21076=CARTESIAN_POINT('Ctrl Pts',(-0.902215926359523,-0.227269801620064,
-0.670378702718353));
#21077=CARTESIAN_POINT('Ctrl Pts',(-0.87482617317514,-0.177024326825049,
-0.705826641853758));
#21078=CARTESIAN_POINT('Ctrl Pts',(-0.861652925570091,-0.144299303100741,
-0.721590372101268));
#21079=CARTESIAN_POINT('Ctrl Pts',(-0.848766861100456,-0.0928409665394229,
-0.736604687327351));
#21080=CARTESIAN_POINT('Ctrl Pts',(-0.84559647055299,-0.0762225747374255,
-0.740223768851063));
#21081=CARTESIAN_POINT('Ctrl Pts',(-0.843383895613249,-0.0595300000000001,
-0.742736168477219));
#21082=CARTESIAN_POINT('',(-0.536443649899847,-0.05953,-0.987512846410683));
#21083=CARTESIAN_POINT('Origin',(0.,-0.05953,0.));
#21084=CARTESIAN_POINT('',(0.0548532617164172,-0.05953,-1.12247250791415));
#21085=CARTESIAN_POINT('Ctrl Pts',(-0.536443649899848,-0.0595300000000001,
-0.987512846410683));
#21086=CARTESIAN_POINT('Ctrl Pts',(-0.533501897135712,-0.0762225747374254,
-0.989110885965947));
#21087=CARTESIAN_POINT('Ctrl Pts',(-0.529268075276156,-0.0928409665394227,
-0.991396466802469));
#21088=CARTESIAN_POINT('Ctrl Pts',(-0.511762781179147,-0.144299303100741,
-1.00061845128527));
#21089=CARTESIAN_POINT('Ctrl Pts',(-0.493462957200432,-0.177024326825049,
-1.0099536580922));
#21090=CARTESIAN_POINT('Ctrl Pts',(-0.45280897844858,-0.227269801620063,
-1.02876878445619));
#21091=CARTESIAN_POINT('Ctrl Pts',(-0.425554672694337,-0.251265615809407,
-1.04048957871266));
#21092=CARTESIAN_POINT('Ctrl Pts',(-0.3787731215897,-0.279889827963178,
-1.05829506364875));
#21093=CARTESIAN_POINT('Ctrl Pts',(-0.354166711873529,-0.290879136862659,
-1.06688848765783));
#21094=CARTESIAN_POINT('Ctrl Pts',(-0.302426893214944,-0.305251990234488,
-1.08269251410343));
#21095=CARTESIAN_POINT('Ctrl Pts',(-0.275287440920027,-0.308638795020976,
-1.0898803575765));
#21096=CARTESIAN_POINT('Ctrl Pts',(-0.224855950742601,-0.308638795020976,
-1.10139101611326));
#21097=CARTESIAN_POINT('Ctrl Pts',(-0.19728546073067,-0.305251990234488,
-1.10669035995599));
#21098=CARTESIAN_POINT('Ctrl Pts',(-0.143812384801039,-0.290879136862659,
-1.11490049012186));
#21099=CARTESIAN_POINT('Ctrl Pts',(-0.117914228755037,-0.279889827963178,
-1.1178344036749));
#21100=CARTESIAN_POINT('Ctrl Pts',(-0.0680399972366989,-0.251265615809407,
-1.12208997038458));
#21101=CARTESIAN_POINT('Ctrl Pts',(-0.0383992541984084,-0.227269801620063,
-1.12335509974011));
#21102=CARTESIAN_POINT('Ctrl Pts',(0.00639229239215326,-0.177024326825049,
-1.12404235695137));
#21103=CARTESIAN_POINT('Ctrl Pts',(0.0269302585198977,-0.144299303100741,
-1.12357162229597));
#21104=CARTESIAN_POINT('Ctrl Pts',(0.04670325263426,-0.0928409665394228,
-1.12285816383385));
#21105=CARTESIAN_POINT('Ctrl Pts',(0.0515094706813703,-0.0762225747374255,
-1.12263591311425));
#21106=CARTESIAN_POINT('Ctrl Pts',(0.0548532617164176,-0.0595300000000001,
-1.12247250791414));
#21107=CARTESIAN_POINT('',(0.437601487681057,-0.05953,-1.03511272300331));
#21108=CARTESIAN_POINT('Origin',(0.,-0.05953,0.));
#21109=CARTESIAN_POINT('',(0.911784794170997,-0.05953,-0.656964154625313));
#21110=CARTESIAN_POINT('Ctrl Pts',(0.437601487681056,-0.0595300000000001,
-1.03511272300331));
#21111=CARTESIAN_POINT('Ctrl Pts',(0.440685038163619,-0.0762225747374255,
-1.03380912944435));
#21112=CARTESIAN_POINT('Ctrl Pts',(0.445111721969657,-0.0928409665394228,
-1.03192403056628));
#21113=CARTESIAN_POINT('Ctrl Pts',(0.463236132117164,-0.144299303100741,
-1.0239876538093));
#21114=CARTESIAN_POINT('Ctrl Pts',(0.481944444320713,-0.177024326825049,
-1.01550068154148));
#21115=CARTESIAN_POINT('Ctrl Pts',(0.522002043615455,-0.227269801620064,
-0.995447160474328));
#21116=CARTESIAN_POINT('Ctrl Pts',(0.548158511259203,-0.251265615809407,
-0.981446681891443));
#21117=CARTESIAN_POINT('Ctrl Pts',(0.591247219971725,-0.279889827963178,
-0.955972930713954));
#21118=CARTESIAN_POINT('Ctrl Pts',(0.613307674922609,-0.290879136862659,
-0.942092777160053));
#21119=CARTESIAN_POINT('Ctrl Pts',(0.657923009631182,-0.305251990234487,
-0.91149460735272));
#21120=CARTESIAN_POINT('Ctrl Pts',(0.680463863683393,-0.308638795020976,
-0.894757676234429));
#21121=CARTESIAN_POINT('Ctrl Pts',(0.720906778729542,-0.308638795020976,
-0.862505527716294));
#21122=CARTESIAN_POINT('Ctrl Pts',(0.742239891936899,-0.305251990234488,
-0.844254137480381));
#21123=CARTESIAN_POINT('Ctrl Pts',(0.781998747691872,-0.290879136862659,
-0.80756613568454));
#21124=CARTESIAN_POINT('Ctrl Pts',(0.800439809856112,-0.279889827963178,
-0.789147407129765));
#21125=CARTESIAN_POINT('Ctrl Pts',(0.834863020612702,-0.251265615809407,
-0.752807465209441));
#21126=CARTESIAN_POINT('Ctrl Pts',(0.854332839576145,-0.227269801620064,
-0.73042219438957));
#21127=CARTESIAN_POINT('Ctrl Pts',(0.882797231409153,-0.177024326825049,
-0.695831250979106));
#21128=CARTESIAN_POINT('Ctrl Pts',(0.895234408667242,-0.144299303100741,
-0.679480524217551));
#21129=CARTESIAN_POINT('Ctrl Pts',(0.907004864562642,-0.0928409665394228,
-0.663576540841106));
#21130=CARTESIAN_POINT('Ctrl Pts',(0.909827729890942,-0.0762225747374256,
-0.659680317203144));
#21131=CARTESIAN_POINT('Ctrl Pts',(0.911784794170998,-0.0595300000000001,
-0.656964154625312));
#21132=CARTESIAN_POINT('',(1.08212377959455,-0.05953,-0.303251606722892));
#21133=CARTESIAN_POINT('Origin',(0.,-0.05953,0.));
#21134=CARTESIAN_POINT('',(1.08212377959455,-0.05953,0.303251606722892));
#21135=CARTESIAN_POINT('Ctrl Pts',(1.08212377959455,-0.0595300000000001,
-0.303251606722892));
#21136=CARTESIAN_POINT('Ctrl Pts',(1.0830271513892,-0.0762225747374255,
-0.300028012588062));
#21137=CARTESIAN_POINT('Ctrl Pts',(1.08431331394788,-0.0928409665394228,
-0.2953917518996));
#21138=CARTESIAN_POINT('Ctrl Pts',(1.08940878963422,-0.144299303100741,
-0.276273267473431));
#21139=CARTESIAN_POINT('Ctrl Pts',(1.09443784939331,-0.177024326825049,
-0.256354979351213));
#21140=CARTESIAN_POINT('Ctrl Pts',(1.10373487993589,-0.227269801620064,
-0.212533521233765));
#21141=CARTESIAN_POINT('Ctrl Pts',(1.10909715583869,-0.251265615809407,
-0.183354415742157));
#21142=CARTESIAN_POINT('Ctrl Pts',(1.1160463456491,-0.279889827963178,-0.133783682657561));
#21143=CARTESIAN_POINT('Ctrl Pts',(1.11894887330541,-0.290879136862659,
-0.107881990270302));
#21144=CARTESIAN_POINT('Ctrl Pts',(1.12284346704144,-0.305251990234488,
-0.0539226701638766));
#21145=CARTESIAN_POINT('Ctrl Pts',(1.123812,-0.308638795020976,-0.025864214957475));
#21146=CARTESIAN_POINT('Ctrl Pts',(1.123812,-0.308638795020976,0.025864214957475));
#21147=CARTESIAN_POINT('Ctrl Pts',(1.12284346704144,-0.305251990234488,
0.0539226701638766));
#21148=CARTESIAN_POINT('Ctrl Pts',(1.11894887330541,-0.290879136862659,
0.107881990270302));
#21149=CARTESIAN_POINT('Ctrl Pts',(1.1160463456491,-0.279889827963178,0.133783682657561));
#21150=CARTESIAN_POINT('Ctrl Pts',(1.10909715583869,-0.251265615809407,
0.183354415742157));
#21151=CARTESIAN_POINT('Ctrl Pts',(1.10373487993589,-0.227269801620064,
0.212533521233765));
#21152=CARTESIAN_POINT('Ctrl Pts',(1.09443784939331,-0.177024326825049,
0.256354979351213));
#21153=CARTESIAN_POINT('Ctrl Pts',(1.08940878963422,-0.144299303100741,
0.276273267473431));
#21154=CARTESIAN_POINT('Ctrl Pts',(1.08431331394788,-0.0928409665394228,
0.2953917518996));
#21155=CARTESIAN_POINT('Ctrl Pts',(1.0830271513892,-0.0762225747374255,
0.300028012588062));
#21156=CARTESIAN_POINT('Ctrl Pts',(1.08212377959455,-0.0595300000000001,
0.303251606722892));
#21157=CARTESIAN_POINT('Origin',(0.,-0.05953,0.));
#21158=CARTESIAN_POINT('Origin',(0.,-0.05953,0.));
#21159=CARTESIAN_POINT('',(0.0589974094846122,-0.05953,1.07456964270265));
#21160=CARTESIAN_POINT('Origin',(0.,-0.05953,0.));
#21161=CARTESIAN_POINT('Origin',(-0.244773027351946,-0.05953,1.07242070340001));
#21162=CARTESIAN_POINT('Origin',(-0.244773027351946,0.,1.07242070340001));
#21163=CARTESIAN_POINT('',(-0.519393123750572,-0.05953,0.942555777842682));
#21164=CARTESIAN_POINT('Ctrl Pts',(-0.519393123750572,-0.05953,0.942555777842682));
#21165=CARTESIAN_POINT('Ctrl Pts',(-0.513714466572041,-0.0925528133349865,
0.945684988399766));
#21166=CARTESIAN_POINT('Ctrl Pts',(-0.503136848051455,-0.124911173756694,
0.951483858396181));
#21167=CARTESIAN_POINT('Ctrl Pts',(-0.47593627990192,-0.177924977804098,
0.965323333309091));
#21168=CARTESIAN_POINT('Ctrl Pts',(-0.460931856495794,-0.199697230012983,
0.972669835243841));
#21169=CARTESIAN_POINT('Ctrl Pts',(-0.426157505475872,-0.237895043532788,
0.988400002689705));
#21170=CARTESIAN_POINT('Ctrl Pts',(-0.406380688682952,-0.254319232363049,
0.996771768218699));
#21171=CARTESIAN_POINT('Ctrl Pts',(-0.364750145543744,-0.28018331644634,
1.01272583306292));
#21172=CARTESIAN_POINT('Ctrl Pts',(-0.340838910881557,-0.29104845371857,
1.02112815447116));
#21173=CARTESIAN_POINT('Ctrl Pts',(-0.290495481564827,-0.30527573347708,
1.036574285215));
#21174=CARTESIAN_POINT('Ctrl Pts',(-0.264056468041074,-0.308638795020976,
1.04359501395068));
#21175=CARTESIAN_POINT('Ctrl Pts',(-0.214892249704082,-0.308638795020976,
1.05481642595959));
#21176=CARTESIAN_POINT('Ctrl Pts',(-0.188025341585962,-0.30527573347708,
1.05996242598502));
#21177=CARTESIAN_POINT('Ctrl Pts',(-0.135965654106109,-0.29104845371857,
1.06788913840721));
#21178=CARTESIAN_POINT('Ctrl Pts',(-0.110776745452494,-0.28018331644634,
1.07069360430242));
#21179=CARTESIAN_POINT('Ctrl Pts',(-0.0663467128214646,-0.254319232363049,
1.07438230428002));
#21180=CARTESIAN_POINT('Ctrl Pts',(-0.0448960436540983,-0.237895043532788,
1.07542044338697));
#21181=CARTESIAN_POINT('Ctrl Pts',(-0.00674037211528124,-0.199697230012983,
1.07633607767727));
#21182=CARTESIAN_POINT('Ctrl Pts',(0.00996567398334777,-0.177924977804098,
1.07622728347683));
#21183=CARTESIAN_POINT('Ctrl Pts',(0.0404772621979741,-0.124911173756694,
1.07556023164702));
#21184=CARTESIAN_POINT('Ctrl Pts',(0.0525234025782719,-0.0925528133349865,
1.07492508698591));
#21185=CARTESIAN_POINT('Ctrl Pts',(0.0589974094846124,-0.05953,1.07456964270265));
#21186=CARTESIAN_POINT('Origin',(-0.244773027351946,-0.05953,1.07242070340001));
#21187=CARTESIAN_POINT('Origin',(0.,-0.05953,0.));
#21188=CARTESIAN_POINT('',(-0.803348093619616,-0.05953,0.716109245731214));
#21189=CARTESIAN_POINT('Origin',(0.,-0.05953,0.));
#21190=CARTESIAN_POINT('Origin',(-0.991065754692661,-0.05953,0.477272113029314));
#21191=CARTESIAN_POINT('Origin',(-0.991065754692661,0.,0.477272113029314));
#21192=CARTESIAN_POINT('',(-1.06075609691358,-0.05953,0.181596019242328));
#21193=CARTESIAN_POINT('Ctrl Pts',(-1.06075609691358,-0.05953,0.181596019242328));
#21194=CARTESIAN_POINT('Ctrl Pts',(-1.05966202740332,-0.0925528133349865,
0.187986803072856));
#21195=CARTESIAN_POINT('Ctrl Pts',(-1.05760072925372,-0.124911173756694,
0.199872254546857));
#21196=CARTESIAN_POINT('Ctrl Pts',(-1.05146158959546,-0.177924977804098,
0.22976728653846));
#21197=CARTESIAN_POINT('Ctrl Pts',(-1.04785021111757,-0.199697230012983,
0.246078686169301));
#21198=CARTESIAN_POINT('Ctrl Pts',(-1.03846709802406,-0.237895043532788,
0.283073967563097));
#21199=CARTESIAN_POINT('Ctrl Pts',(-1.03268176429485,-0.254319232363049,
0.303755815985685));
#21200=CARTESIAN_POINT('Ctrl Pts',(-1.01919893537026,-0.28018331644634,
0.346251081972725));
#21201=CARTESIAN_POINT('Ctrl Pts',(-1.01085972381132,-0.29104845371857,
0.370184399726282));
#21202=CARTESIAN_POINT('Ctrl Pts',(-0.99154738033959,-0.30527573347708,
0.419174982698463));
#21203=CARTESIAN_POINT('Ctrl Pts',(-0.980551951791748,-0.308638795020976,
0.444223188605045));
#21204=CARTESIAN_POINT('Ctrl Pts',(-0.958671816228589,-0.308638795020976,
0.489657758261848));
#21205=CARTESIAN_POINT('Ctrl Pts',(-0.945943877838127,-0.30527573347708,
0.51387163140139));
#21206=CARTESIAN_POINT('Ctrl Pts',(-0.91968254693063,-0.29104845371857,
0.559515758398093));
#21207=CARTESIAN_POINT('Ctrl Pts',(-0.906170138993533,-0.28018331644634,
0.580957796077825));
#21208=CARTESIAN_POINT('Ctrl Pts',(-0.8813524085237,-0.254319232363049,
0.617994461173994));
#21209=CARTESIAN_POINT('Ctrl Pts',(-0.868789784891799,-0.237895043532788,
0.635412538795143));
#21210=CARTESIAN_POINT('Ctrl Pts',(-0.845715984518854,-0.199697230012983,
0.66581473268113));
#21211=CARTESIAN_POINT('Ctrl Pts',(-0.835214876415962,-0.177924977804098,
0.678808213394124));
#21212=CARTESIAN_POINT('Ctrl Pts',(-0.815669690204649,-0.124911173756694,
0.702247233627224));
#21213=CARTESIAN_POINT('Ctrl Pts',(-0.807662468433796,-0.0925528133349865,
0.711269279199861));
#21214=CARTESIAN_POINT('Ctrl Pts',(-0.803348093619616,-0.05953,0.716109245731214));
#21215=CARTESIAN_POINT('Origin',(-0.991065754692661,-0.05953,0.477272113029314));
#21216=CARTESIAN_POINT('Origin',(0.,-0.05953,0.));
#21217=CARTESIAN_POINT('',(-1.076188,-0.05953,1.31795018948079E-16));
#21218=CARTESIAN_POINT('Origin',(0.,-0.05953,0.));
#21219=CARTESIAN_POINT('',(-1.06075609691358,-0.05953,-0.181596019242328));
#21220=CARTESIAN_POINT('Origin',(0.,-0.05953,0.));
#21221=CARTESIAN_POINT('Origin',(-0.991065754692661,-0.05953,-0.477272113029314));
#21222=CARTESIAN_POINT('Origin',(-0.991065754692661,0.,-0.477272113029314));
#21223=CARTESIAN_POINT('',(-0.803348093619616,-0.05953,-0.716109245731215));
#21224=CARTESIAN_POINT('Ctrl Pts',(-0.803348093619616,-0.05953,-0.716109245731215));
#21225=CARTESIAN_POINT('Ctrl Pts',(-0.807662468433795,-0.0925528133349865,
-0.711269279199862));
#21226=CARTESIAN_POINT('Ctrl Pts',(-0.815669690204649,-0.124911173756694,
-0.702247233627224));
#21227=CARTESIAN_POINT('Ctrl Pts',(-0.835214876415962,-0.177924977804098,
-0.678808213394124));
#21228=CARTESIAN_POINT('Ctrl Pts',(-0.845715984518854,-0.199697230012983,
-0.66581473268113));
#21229=CARTESIAN_POINT('Ctrl Pts',(-0.868789784891799,-0.237895043532788,
-0.635412538795143));
#21230=CARTESIAN_POINT('Ctrl Pts',(-0.8813524085237,-0.254319232363049,
-0.617994461173994));
#21231=CARTESIAN_POINT('Ctrl Pts',(-0.906170138993533,-0.28018331644634,
-0.580957796077826));
#21232=CARTESIAN_POINT('Ctrl Pts',(-0.91968254693063,-0.29104845371857,
-0.559515758398093));
#21233=CARTESIAN_POINT('Ctrl Pts',(-0.945943877838127,-0.30527573347708,
-0.51387163140139));
#21234=CARTESIAN_POINT('Ctrl Pts',(-0.958671816228589,-0.308638795020976,
-0.489657758261848));
#21235=CARTESIAN_POINT('Ctrl Pts',(-0.980551951791748,-0.308638795020976,
-0.444223188605045));
#21236=CARTESIAN_POINT('Ctrl Pts',(-0.99154738033959,-0.30527573347708,
-0.419174982698463));
#21237=CARTESIAN_POINT('Ctrl Pts',(-1.01085972381132,-0.29104845371857,
-0.370184399726282));
#21238=CARTESIAN_POINT('Ctrl Pts',(-1.01919893537026,-0.28018331644634,
-0.346251081972725));
#21239=CARTESIAN_POINT('Ctrl Pts',(-1.03268176429485,-0.254319232363049,
-0.303755815985685));
#21240=CARTESIAN_POINT('Ctrl Pts',(-1.03846709802406,-0.237895043532788,
-0.283073967563097));
#21241=CARTESIAN_POINT('Ctrl Pts',(-1.04785021111757,-0.199697230012983,
-0.246078686169302));
#21242=CARTESIAN_POINT('Ctrl Pts',(-1.05146158959546,-0.177924977804098,
-0.229767286538461));
#21243=CARTESIAN_POINT('Ctrl Pts',(-1.05760072925372,-0.124911173756694,
-0.199872254546858));
#21244=CARTESIAN_POINT('Ctrl Pts',(-1.05966202740332,-0.0925528133349864,
-0.187986803072857));
#21245=CARTESIAN_POINT('Ctrl Pts',(-1.06075609691358,-0.05953,-0.181596019242328));
#21246=CARTESIAN_POINT('Origin',(-0.991065754692661,-0.05953,-0.477272113029314));
#21247=CARTESIAN_POINT('Origin',(0.,-0.05953,0.));
#21248=CARTESIAN_POINT('',(-0.519393123750572,-0.05953,-0.942555777842682));
#21249=CARTESIAN_POINT('Origin',(0.,-0.05953,0.));
#21250=CARTESIAN_POINT('Origin',(-0.244773027351946,-0.05953,-1.07242070340001));
#21251=CARTESIAN_POINT('Origin',(-0.244773027351946,0.,-1.07242070340001));
#21252=CARTESIAN_POINT('',(0.0589974094846125,-0.05953,-1.07456964270265));
#21253=CARTESIAN_POINT('Ctrl Pts',(0.0589974094846127,-0.05953,-1.07456964270265));
#21254=CARTESIAN_POINT('Ctrl Pts',(0.0525234025782722,-0.0925528133349865,
-1.07492508698591));
#21255=CARTESIAN_POINT('Ctrl Pts',(0.0404772621979744,-0.124911173756694,
-1.07556023164702));
#21256=CARTESIAN_POINT('Ctrl Pts',(0.0099656739833481,-0.177924977804098,
-1.07622728347683));
#21257=CARTESIAN_POINT('Ctrl Pts',(-0.00674037211528096,-0.199697230012983,
-1.07633607767727));
#21258=CARTESIAN_POINT('Ctrl Pts',(-0.044896043654098,-0.237895043532788,
-1.07542044338697));
#21259=CARTESIAN_POINT('Ctrl Pts',(-0.0663467128214644,-0.254319232363049,
-1.07438230428002));
#21260=CARTESIAN_POINT('Ctrl Pts',(-0.110776745452493,-0.28018331644634,
-1.07069360430242));
#21261=CARTESIAN_POINT('Ctrl Pts',(-0.135965654106109,-0.29104845371857,
-1.06788913840721));
#21262=CARTESIAN_POINT('Ctrl Pts',(-0.188025341585962,-0.30527573347708,
-1.05996242598502));
#21263=CARTESIAN_POINT('Ctrl Pts',(-0.214892249704082,-0.308638795020976,
-1.05481642595959));
#21264=CARTESIAN_POINT('Ctrl Pts',(-0.264056468041074,-0.308638795020976,
-1.04359501395068));
#21265=CARTESIAN_POINT('Ctrl Pts',(-0.290495481564827,-0.30527573347708,
-1.036574285215));
#21266=CARTESIAN_POINT('Ctrl Pts',(-0.340838910881557,-0.291048453718569,
-1.02112815447116));
#21267=CARTESIAN_POINT('Ctrl Pts',(-0.364750145543744,-0.28018331644634,
-1.01272583306292));
#21268=CARTESIAN_POINT('Ctrl Pts',(-0.406380688682952,-0.254319232363049,
-0.996771768218699));
#21269=CARTESIAN_POINT('Ctrl Pts',(-0.426157505475872,-0.237895043532788,
-0.988400002689705));
#21270=CARTESIAN_POINT('Ctrl Pts',(-0.460931856495794,-0.199697230012983,
-0.972669835243841));
#21271=CARTESIAN_POINT('Ctrl Pts',(-0.475936279901919,-0.177924977804098,
-0.965323333309091));
#21272=CARTESIAN_POINT('Ctrl Pts',(-0.503136848051454,-0.124911173756694,
-0.951483858396181));
#21273=CARTESIAN_POINT('Ctrl Pts',(-0.513714466572041,-0.0925528133349865,
-0.945684988399766));
#21274=CARTESIAN_POINT('Ctrl Pts',(-0.519393123750572,-0.05953,-0.942555777842682));
#21275=CARTESIAN_POINT('Origin',(-0.244773027351946,-0.05953,-1.07242070340001));
#21276=CARTESIAN_POINT('Origin',(0.,-0.05953,0.));
#21277=CARTESIAN_POINT('',(0.413083465285518,-0.05953,-0.993751811093549));
#21278=CARTESIAN_POINT('Origin',(0.,-0.05953,0.));
#21279=CARTESIAN_POINT('Origin',(0.685838782044607,-0.05953,-0.860014630714833));
#21280=CARTESIAN_POINT('Origin',(0.685838782044607,0.,-0.860014630714833));
#21281=CARTESIAN_POINT('',(0.876916659919095,-0.05953,-0.623857181492959));
#21282=CARTESIAN_POINT('Ctrl Pts',(0.876916659919095,-0.05953,-0.623857181492958));
#21283=CARTESIAN_POINT('Ctrl Pts',(0.873158080166742,-0.0925528133349865,
-0.62914037979579));
#21284=CARTESIAN_POINT('Ctrl Pts',(0.866144010579847,-0.124911173756694,
-0.638954437806245));
#21285=CARTESIAN_POINT('Ctrl Pts',(0.847641868610495,-0.177924977804098,
-0.663225258065736));
#21286=CARTESIAN_POINT('Ctrl Pts',(0.837310877969633,-0.199697230012983,
-0.676354402927683));
#21287=CARTESIAN_POINT('Ctrl Pts',(0.81280533416753,-0.237895043532788,
-0.705614819529209));
#21288=CARTESIAN_POINT('Ctrl Pts',(0.798619410861634,-0.254319232363049,
-0.721738358858166));
#21289=CARTESIAN_POINT('Ctrl Pts',(0.768033796848072,-0.28018331644634,
-0.754175290318038));
#21290=CARTESIAN_POINT('Ctrl Pts',(0.750136149454208,-0.29104845371857,
-0.772120216227122));
#21291=CARTESIAN_POINT('Ctrl Pts',(0.711480111898423,-0.30527573347708,
-0.807879894508811));
#21292=CARTESIAN_POINT('Ctrl Pts',(0.690705563850638,-0.308638795020976,
-0.825676810575913));
#21293=CARTESIAN_POINT('Ctrl Pts',(0.651278921914856,-0.308638795020976,
-0.857118508332695));
#21294=CARTESIAN_POINT('Ctrl Pts',(0.629305439856167,-0.30527573347708,
-0.873412008702649));
#21295=CARTESIAN_POINT('Ctrl Pts',(0.585840553788742,-0.29104845371857,
-0.903141581680914));
#21296=CARTESIAN_POINT('Ctrl Pts',(0.564362943424239,-0.28018331644634,
-0.916597376014514));
#21297=CARTESIAN_POINT('Ctrl Pts',(0.525933334162556,-0.254319232363049,
-0.939198248544427));
#21298=CARTESIAN_POINT('Ctrl Pts',(0.507057380724533,-0.237895043532788,
-0.949440676105255));
#21299=CARTESIAN_POINT('Ctrl Pts',(0.473077587363686,-0.199697230012983,
-0.966820759530997));
#21300=CARTESIAN_POINT('Ctrl Pts',(0.457978755888596,-0.177924977804098,
-0.973971221090534));
#21301=CARTESIAN_POINT('Ctrl Pts',(0.430199341854858,-0.124911173756694,
-0.986608710139579));
#21302=CARTESIAN_POINT('Ctrl Pts',(0.419070565453384,-0.0925528133349865,
-0.991263089003441));
#21303=CARTESIAN_POINT('Ctrl Pts',(0.413083465285518,-0.05953,-0.993751811093549));
#21304=CARTESIAN_POINT('Origin',(0.685838782044607,-0.05953,-0.860014630714833));
#21305=CARTESIAN_POINT('Origin',(0.,-0.208355,0.));
#21306=CARTESIAN_POINT('',(-1.076188,-0.35718,1.31795018948079E-16));
#21307=CARTESIAN_POINT('Origin',(0.,-0.35718,0.));
#21308=CARTESIAN_POINT('',(-1.076188,-0.208355,1.31795018948079E-16));
#21309=CARTESIAN_POINT('',(1.03449977959455,-0.05953,0.296632461748266));
#21310=CARTESIAN_POINT('Origin',(0.,-0.05953,0.));
#21311=CARTESIAN_POINT('',(1.03449977959455,-0.05953,-0.296632461748266));
#21312=CARTESIAN_POINT('Ctrl Pts',(1.03449977959455,-0.05953,0.296632461748267));
#21313=CARTESIAN_POINT('Ctrl Pts',(1.03628691421076,-0.0925528133349865,
0.290399865505497));
#21314=CARTESIAN_POINT('Ctrl Pts',(1.03958665287714,-0.124911173756694,
0.278797079997872));
#21315=CARTESIAN_POINT('Ctrl Pts',(1.0470264474309,-0.177924977804098,0.249198913998601));
#21316=CARTESIAN_POINT('Ctrl Pts',(1.05084995891418,-0.199697230012983,
0.232935932341942));
#21317=CARTESIAN_POINT('Ctrl Pts',(1.05844771715377,-0.237895043532788,
0.195533155353269));
#21318=CARTESIAN_POINT('Ctrl Pts',(1.06220882929878,-0.254319232363049,
0.17438929156337));
#21319=CARTESIAN_POINT('Ctrl Pts',(1.06849922508772,-0.28018331644634,0.130252399648131));
#21320=CARTESIAN_POINT('Ctrl Pts',(1.07137013248666,-0.29104845371857,0.105070977154072));
#21321=CARTESIAN_POINT('Ctrl Pts',(1.07522652957392,-0.30527573347708,0.0525526752791107));
#21322=CARTESIAN_POINT('Ctrl Pts',(1.076188,-0.308638795020976,0.025214283908933));
#21323=CARTESIAN_POINT('Ctrl Pts',(1.076188,-0.308638795020976,-0.025214283908933));
#21324=CARTESIAN_POINT('Ctrl Pts',(1.07522652957392,-0.30527573347708,-0.0525526752791107));
#21325=CARTESIAN_POINT('Ctrl Pts',(1.07137013248666,-0.29104845371857,-0.105070977154072));
#21326=CARTESIAN_POINT('Ctrl Pts',(1.06849922508772,-0.28018331644634,-0.130252399648131));
#21327=CARTESIAN_POINT('Ctrl Pts',(1.06220882929878,-0.254319232363049,
-0.17438929156337));
#21328=CARTESIAN_POINT('Ctrl Pts',(1.05844771715377,-0.237895043532788,
-0.195533155353269));
#21329=CARTESIAN_POINT('Ctrl Pts',(1.05084995891418,-0.199697230012983,
-0.232935932341942));
#21330=CARTESIAN_POINT('Ctrl Pts',(1.0470264474309,-0.177924977804098,-0.249198913998601));
#21331=CARTESIAN_POINT('Ctrl Pts',(1.03958665287714,-0.124911173756694,
-0.278797079997872));
#21332=CARTESIAN_POINT('Ctrl Pts',(1.03628691421076,-0.0925528133349865,
-0.290399865505497));
#21333=CARTESIAN_POINT('Ctrl Pts',(1.03449977959455,-0.05953,-0.296632461748267));
#21334=CARTESIAN_POINT('Origin',(0.,-0.05953,0.));
#21335=CARTESIAN_POINT('Origin',(0.,-0.05953,0.));
#21336=CARTESIAN_POINT('Origin',(1.1,-0.05953,0.));
#21337=CARTESIAN_POINT('Origin',(1.1,0.,0.));
#21338=CARTESIAN_POINT('Origin',(1.1,-0.05953,0.));
#21339=CARTESIAN_POINT('Origin',(0.,-0.35718,0.));
#21340=CARTESIAN_POINT('Origin',(0.,-0.05953,0.));
#23498=UNCERTAINTY_MEASURE_WITH_UNIT(LENGTH_MEASURE(0.001),#23588,
'DISTANCE_ACCURACY_VALUE',
'Maximum model space distance between geometric entities at asserted c
onnectivities');
#23522=UNCERTAINTY_MEASURE_WITH_UNIT(LENGTH_MEASURE(0.001),#23588,
'DISTANCE_ACCURACY_VALUE',
'Maximum model space distance between geometric entities at asserted c
onnectivities');
#23563=(
GEOMETRIC_REPRESENTATION_CONTEXT(3)
GLOBAL_UNCERTAINTY_ASSIGNED_CONTEXT((#23498))
GLOBAL_UNIT_ASSIGNED_CONTEXT((#23588,#23590,#23591))
REPRESENTATION_CONTEXT('','3D')
);
#23587=(
GEOMETRIC_REPRESENTATION_CONTEXT(3)
GLOBAL_UNCERTAINTY_ASSIGNED_CONTEXT((#23522))
GLOBAL_UNIT_ASSIGNED_CONTEXT((#23588,#23590,#23591))
REPRESENTATION_CONTEXT('','3D')
);
#23588=(
LENGTH_UNIT()
NAMED_UNIT(*)
SI_UNIT(.CENTI.,.METRE.)
);
#23590=(
NAMED_UNIT(*)
PLANE_ANGLE_UNIT()
SI_UNIT($,.RADIAN.)
);
#23591=(
NAMED_UNIT(*)
SI_UNIT($,.STERADIAN.)
SOLID_ANGLE_UNIT()
);
#23632=SHAPE_DEFINITION_REPRESENTATION(#23704,#23865);
#23704=PRODUCT_DEFINITION_SHAPE('',$,#23930);
#23865=SHAPE_REPRESENTATION('',(#13709),#23563);
#23889=PRODUCT_DEFINITION_CONTEXT('part definition',#24083,'design');
#23930=PRODUCT_DEFINITION('Cage (1)','Cage (1)',#23994,#23889);
#23994=PRODUCT_DEFINITION_FORMATION('',$,#24125);
#24083=APPLICATION_CONTEXT(
'Core Data for Automotive Mechanical Design Process');
#24084=PRODUCT_CONTEXT('part definition',#24083,'mechanical');
#24125=PRODUCT('Cage (1)','Cage (1)','Cage (1)',(#24084));
#24205=COLOUR_RGB('Grey',0.48,0.52,0.57);
#24206=FILL_AREA_STYLE_COLOUR('',#24205);
#24207=FILL_AREA_STYLE('',(#24206));
#24208=SURFACE_STYLE_FILL_AREA(#24207);
#24209=SURFACE_SIDE_STYLE('',(#24208));
#24210=SURFACE_STYLE_USAGE(.BOTH.,#24209);
#24211=PRESENTATION_STYLE_ASSIGNMENT((#24210));
ENDSEC;
END-ISO-10303-21;
